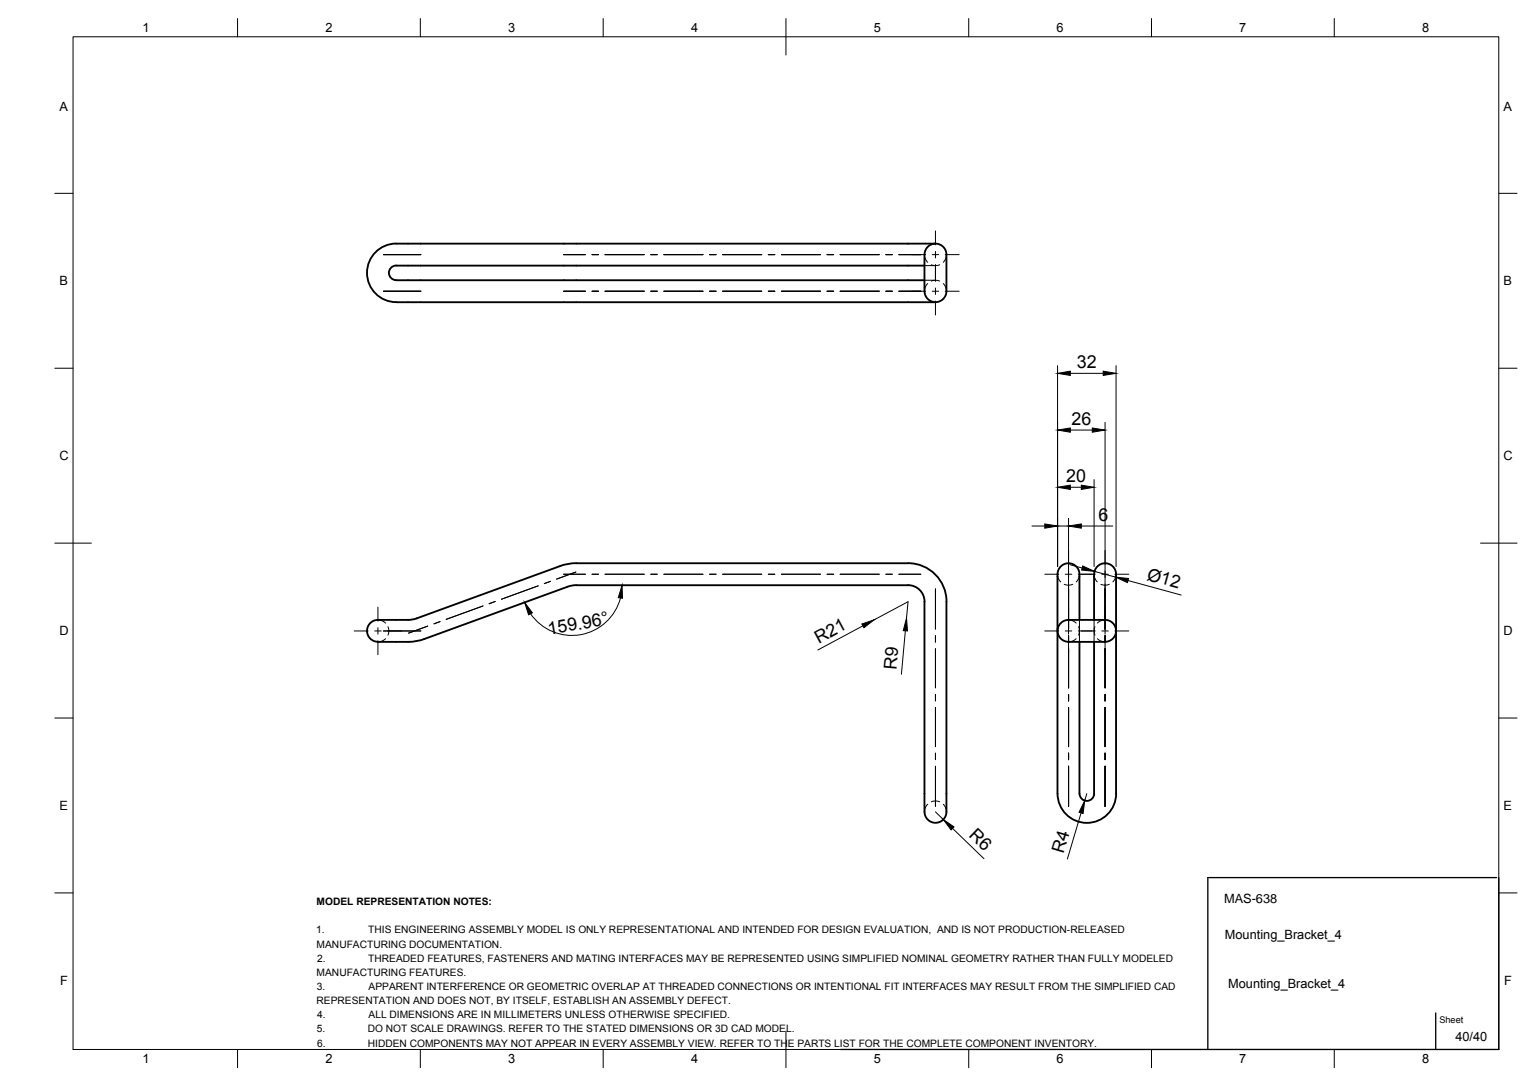
ISO-10303-21;
HEADER;
FILE_DESCRIPTION((''),'2;1');
FILE_NAME('Mounting_Bracket_4.step','2026-10-09T12:00:21-07:00',(''),(''),'','','');
FILE_SCHEMA (('AUTOMOTIVE_DESIGN { 1 0 10303 214 3 1 1 }'));
ENDSEC;
DATA;
#10=MECHANICAL_DESIGN_GEOMETRIC_PRESENTATION_REPRESENTATION('',(#435),#10334);
#184=CYLINDRICAL_SURFACE('',#4428,0.600000000000001) ;
#185=CYLINDRICAL_SURFACE('',#4429,0.600000000000001) ;
#186=CYLINDRICAL_SURFACE('',#4430,0.599999999999996) ;
#187=CYLINDRICAL_SURFACE('',#4431,0.600000000000001) ;
#188=CYLINDRICAL_SURFACE('',#4432,0.600000000000001) ;
#189=CYLINDRICAL_SURFACE('',#4433,0.600000000000001) ;
#190=CYLINDRICAL_SURFACE('',#4434,0.599999999999996) ;
#191=CYLINDRICAL_SURFACE('',#4435,0.600000000000001) ;
#363=SHAPE_REPRESENTATION_RELATIONSHIP('SRR','None',#10481,#395) ;
#395=ADVANCED_BREP_SHAPE_REPRESENTATION('',(#467),#10333) ;
#435=STYLED_ITEM('',(#10631),#467) ;
#467=MANIFOLD_SOLID_BREP('Body1',#3589) ;
#682=LINE('',#10238,#840) ;
#683=LINE('',#10240,#841) ;
#684=LINE('',#10242,#842) ;
#685=LINE('',#10244,#843) ;
#686=LINE('',#10246,#844) ;
#687=LINE('',#10248,#845) ;
#688=LINE('',#10250,#846) ;
#689=LINE('',#10252,#847) ;
#840=VECTOR('',#5566,0.600000000000001) ;
#841=VECTOR('',#5569,0.600000000000001) ;
#842=VECTOR('',#5572,0.599999999999996) ;
#843=VECTOR('',#5575,0.600000000000001) ;
#844=VECTOR('',#5578,0.600000000000001) ;
#845=VECTOR('',#5581,0.600000000000001) ;
#846=VECTOR('',#5584,0.599999999999996) ;
#847=VECTOR('',#5587,0.600000000000001) ;
#1034=FACE_OUTER_BOUND('',#1242,.T.) ;
#1035=FACE_OUTER_BOUND('',#1243,.T.) ;
#1036=FACE_OUTER_BOUND('',#1244,.T.) ;
#1037=FACE_OUTER_BOUND('',#1245,.T.) ;
#1038=FACE_OUTER_BOUND('',#1246,.T.) ;
#1039=FACE_OUTER_BOUND('',#1247,.T.) ;
#1040=FACE_OUTER_BOUND('',#1248,.T.) ;
#1041=FACE_OUTER_BOUND('',#1249,.T.) ;
#1042=FACE_OUTER_BOUND('',#1250,.T.) ;
#1043=FACE_OUTER_BOUND('',#1251,.T.) ;
#1044=FACE_OUTER_BOUND('',#1252,.T.) ;
#1045=FACE_OUTER_BOUND('',#1253,.T.) ;
#1046=FACE_OUTER_BOUND('',#1254,.T.) ;
#1047=FACE_OUTER_BOUND('',#1255,.T.) ;
#1048=FACE_OUTER_BOUND('',#1256,.T.) ;
#1049=FACE_OUTER_BOUND('',#1257,.T.) ;
#1242=EDGE_LOOP('',(#3217,#3218,#3219,#3220,#3221)) ;
#1243=EDGE_LOOP('',(#3222,#3223,#3224,#3225)) ;
#1244=EDGE_LOOP('',(#3226,#3227,#3228,#3229,#3230,#3231)) ;
#1245=EDGE_LOOP('',(#3232,#3233,#3234,#3235,#3236,#3237)) ;
#1246=EDGE_LOOP('',(#3238,#3239,#3240,#3241,#3242,#3243)) ;
#1247=EDGE_LOOP('',(#3244,#3245,#3246,#3247,#3248)) ;
#1248=EDGE_LOOP('',(#3249,#3250,#3251,#3252)) ;
#1249=EDGE_LOOP('',(#3253,#3254,#3255,#3256,#3257,#3258)) ;
#1250=EDGE_LOOP('',(#3259,#3260,#3261,#3262,#3263,#3264)) ;
#1251=EDGE_LOOP('',(#3265,#3266,#3267,#3268)) ;
#1252=EDGE_LOOP('',(#3269,#3270,#3271,#3272,#3273)) ;
#1253=EDGE_LOOP('',(#3274,#3275,#3276,#3277,#3278,#3279)) ;
#1254=EDGE_LOOP('',(#3280,#3281,#3282,#3283,#3284,#3285)) ;
#1255=EDGE_LOOP('',(#3286,#3287,#3288,#3289)) ;
#1256=EDGE_LOOP('',(#3290,#3291,#3292,#3293,#3294)) ;
#1257=EDGE_LOOP('',(#3295,#3296,#3297,#3298,#3299,#3300)) ;
#1465=CIRCLE('',#4387,0.600000000000001) ;
#1466=CIRCLE('',#4388,0.899999999999999) ;
#1467=CIRCLE('',#4389,0.600000000000001) ;
#1468=CIRCLE('',#4390,0.600000000000001) ;
#1469=CIRCLE('',#4392,0.600000000000001) ;
#1470=CIRCLE('',#4393,1.4) ;
#1471=CIRCLE('',#4394,0.600000000000001) ;
#1472=CIRCLE('',#4396,0.600000000000001) ;
#1473=CIRCLE('',#4397,0.600000000000001) ;
#1474=CIRCLE('',#4398,1.4) ;
#1475=CIRCLE('',#4399,0.600000000000001) ;
#1476=CIRCLE('',#4400,0.600000000000001) ;
#1477=CIRCLE('',#4402,0.600000000000001) ;
#1478=CIRCLE('',#4403,0.399999999999999) ;
#1479=CIRCLE('',#4404,0.600000000000001) ;
#1480=CIRCLE('',#4405,0.600000000000001) ;
#1481=CIRCLE('',#4406,0.600000000000001) ;
#1482=CIRCLE('',#4408,0.600000000000001) ;
#1483=CIRCLE('',#4409,0.600000000000001) ;
#1484=CIRCLE('',#4410,0.400000000000002) ;
#1485=CIRCLE('',#4411,0.600000000000001) ;
#1486=CIRCLE('',#4412,0.600000000000001) ;
#1487=CIRCLE('',#4414,0.600000000000001) ;
#1488=CIRCLE('',#4415,0.600000000000001) ;
#1489=CIRCLE('',#4416,0.899999999999999) ;
#1490=CIRCLE('',#4417,0.600000000000001) ;
#1491=CIRCLE('',#4419,0.600000000000001) ;
#1492=CIRCLE('',#4420,1.4) ;
#1493=CIRCLE('',#4421,0.600000000000001) ;
#1494=CIRCLE('',#4423,0.600000000000001) ;
#1495=CIRCLE('',#4424,0.600000000000001) ;
#1496=CIRCLE('',#4425,1.4) ;
#1497=CIRCLE('',#4426,0.600000000000001) ;
#1498=CIRCLE('',#4427,0.600000000000001) ;
#1784=VERTEX_POINT('',#10170) ;
#1785=VERTEX_POINT('',#10172) ;
#1786=VERTEX_POINT('',#10174) ;
#1787=VERTEX_POINT('',#10178) ;
#1788=VERTEX_POINT('',#10180) ;
#1789=VERTEX_POINT('',#10184) ;
#1790=VERTEX_POINT('',#10185) ;
#1791=VERTEX_POINT('',#10188) ;
#1792=VERTEX_POINT('',#10190) ;
#1793=VERTEX_POINT('',#10194) ;
#1794=VERTEX_POINT('',#10195) ;
#1795=VERTEX_POINT('',#10197) ;
#1796=VERTEX_POINT('',#10199) ;
#1797=VERTEX_POINT('',#10204) ;
#1798=VERTEX_POINT('',#10205) ;
#1799=VERTEX_POINT('',#10208) ;
#1800=VERTEX_POINT('',#10210) ;
#1801=VERTEX_POINT('',#10214) ;
#1802=VERTEX_POINT('',#10215) ;
#1803=VERTEX_POINT('',#10218) ;
#1804=VERTEX_POINT('',#10222) ;
#1805=VERTEX_POINT('',#10224) ;
#1806=VERTEX_POINT('',#10228) ;
#1807=VERTEX_POINT('',#10229) ;
#1808=VERTEX_POINT('',#10232) ;
#1809=VERTEX_POINT('',#10234) ;
#2265=EDGE_CURVE('',#1784,#1784,#1465,.T.) ;
#2266=EDGE_CURVE('',#1784,#1785,#1466,.T.) ;
#2267=EDGE_CURVE('',#1785,#1786,#1467,.T.) ;
#2268=EDGE_CURVE('',#1786,#1785,#1468,.T.) ;
#2269=EDGE_CURVE('',#1787,#1787,#1469,.T.) ;
#2270=EDGE_CURVE('',#1787,#1788,#1470,.T.) ;
#2271=EDGE_CURVE('',#1788,#1788,#1471,.T.) ;
#2272=EDGE_CURVE('',#1789,#1790,#1472,.T.) ;
#2273=EDGE_CURVE('',#1790,#1789,#1473,.T.) ;
#2274=EDGE_CURVE('',#1790,#1791,#1474,.T.) ;
#2275=EDGE_CURVE('',#1791,#1792,#1475,.T.) ;
#2276=EDGE_CURVE('',#1792,#1791,#1476,.T.) ;
#2277=EDGE_CURVE('',#1793,#1794,#1477,.T.) ;
#2278=EDGE_CURVE('',#1794,#1795,#1478,.T.) ;
#2279=EDGE_CURVE('',#1796,#1795,#1479,.T.) ;
#2280=EDGE_CURVE('',#1795,#1796,#1480,.T.) ;
#2281=EDGE_CURVE('',#1794,#1793,#1481,.T.) ;
#2282=EDGE_CURVE('',#1797,#1798,#1482,.T.) ;
#2283=EDGE_CURVE('',#1798,#1797,#1483,.T.) ;
#2284=EDGE_CURVE('',#1798,#1799,#1484,.T.) ;
#2285=EDGE_CURVE('',#1799,#1800,#1485,.T.) ;
#2286=EDGE_CURVE('',#1800,#1799,#1486,.T.) ;
#2287=EDGE_CURVE('',#1801,#1802,#1487,.T.) ;
#2288=EDGE_CURVE('',#1802,#1801,#1488,.T.) ;
#2289=EDGE_CURVE('',#1802,#1803,#1489,.T.) ;
#2290=EDGE_CURVE('',#1803,#1803,#1490,.T.) ;
#2291=EDGE_CURVE('',#1804,#1804,#1491,.T.) ;
#2292=EDGE_CURVE('',#1804,#1805,#1492,.T.) ;
#2293=EDGE_CURVE('',#1805,#1805,#1493,.T.) ;
#2294=EDGE_CURVE('',#1806,#1807,#1494,.T.) ;
#2295=EDGE_CURVE('',#1807,#1806,#1495,.T.) ;
#2296=EDGE_CURVE('',#1807,#1808,#1496,.T.) ;
#2297=EDGE_CURVE('',#1808,#1809,#1497,.T.) ;
#2298=EDGE_CURVE('',#1809,#1808,#1498,.T.) ;
#2299=EDGE_CURVE('',#1797,#1786,#682,.T.) ;
#2300=EDGE_CURVE('',#1784,#1788,#683,.T.) ;
#2301=EDGE_CURVE('',#1787,#1792,#684,.T.) ;
#2302=EDGE_CURVE('',#1789,#1793,#685,.T.) ;
#2303=EDGE_CURVE('',#1800,#1801,#686,.T.) ;
#2304=EDGE_CURVE('',#1803,#1804,#687,.T.) ;
#2305=EDGE_CURVE('',#1805,#1806,#688,.T.) ;
#2306=EDGE_CURVE('',#1809,#1796,#689,.T.) ;
#3217=ORIENTED_EDGE('',*,*,#2265,.F.) ;
#3218=ORIENTED_EDGE('',*,*,#2266,.T.) ;
#3219=ORIENTED_EDGE('',*,*,#2267,.T.) ;
#3220=ORIENTED_EDGE('',*,*,#2268,.T.) ;
#3221=ORIENTED_EDGE('',*,*,#2266,.F.) ;
#3222=ORIENTED_EDGE('',*,*,#2269,.F.) ;
#3223=ORIENTED_EDGE('',*,*,#2270,.T.) ;
#3224=ORIENTED_EDGE('',*,*,#2271,.T.) ;
#3225=ORIENTED_EDGE('',*,*,#2270,.F.) ;
#3226=ORIENTED_EDGE('',*,*,#2272,.F.) ;
#3227=ORIENTED_EDGE('',*,*,#2273,.F.) ;
#3228=ORIENTED_EDGE('',*,*,#2274,.T.) ;
#3229=ORIENTED_EDGE('',*,*,#2275,.T.) ;
#3230=ORIENTED_EDGE('',*,*,#2276,.T.) ;
#3231=ORIENTED_EDGE('',*,*,#2274,.F.) ;
#3232=ORIENTED_EDGE('',*,*,#2277,.T.) ;
#3233=ORIENTED_EDGE('',*,*,#2278,.T.) ;
#3234=ORIENTED_EDGE('',*,*,#2279,.F.) ;
#3235=ORIENTED_EDGE('',*,*,#2280,.F.) ;
#3236=ORIENTED_EDGE('',*,*,#2278,.F.) ;
#3237=ORIENTED_EDGE('',*,*,#2281,.T.) ;
#3238=ORIENTED_EDGE('',*,*,#2282,.F.) ;
#3239=ORIENTED_EDGE('',*,*,#2283,.F.) ;
#3240=ORIENTED_EDGE('',*,*,#2284,.T.) ;
#3241=ORIENTED_EDGE('',*,*,#2285,.T.) ;
#3242=ORIENTED_EDGE('',*,*,#2286,.T.) ;
#3243=ORIENTED_EDGE('',*,*,#2284,.F.) ;
#3244=ORIENTED_EDGE('',*,*,#2287,.F.) ;
#3245=ORIENTED_EDGE('',*,*,#2288,.F.) ;
#3246=ORIENTED_EDGE('',*,*,#2289,.T.) ;
#3247=ORIENTED_EDGE('',*,*,#2290,.T.) ;
#3248=ORIENTED_EDGE('',*,*,#2289,.F.) ;
#3249=ORIENTED_EDGE('',*,*,#2291,.F.) ;
#3250=ORIENTED_EDGE('',*,*,#2292,.T.) ;
#3251=ORIENTED_EDGE('',*,*,#2293,.T.) ;
#3252=ORIENTED_EDGE('',*,*,#2292,.F.) ;
#3253=ORIENTED_EDGE('',*,*,#2294,.F.) ;
#3254=ORIENTED_EDGE('',*,*,#2295,.F.) ;
#3255=ORIENTED_EDGE('',*,*,#2296,.T.) ;
#3256=ORIENTED_EDGE('',*,*,#2297,.T.) ;
#3257=ORIENTED_EDGE('',*,*,#2298,.T.) ;
#3258=ORIENTED_EDGE('',*,*,#2296,.F.) ;
#3259=ORIENTED_EDGE('',*,*,#2282,.T.) ;
#3260=ORIENTED_EDGE('',*,*,#2283,.T.) ;
#3261=ORIENTED_EDGE('',*,*,#2299,.T.) ;
#3262=ORIENTED_EDGE('',*,*,#2267,.F.) ;
#3263=ORIENTED_EDGE('',*,*,#2268,.F.) ;
#3264=ORIENTED_EDGE('',*,*,#2299,.F.) ;
#3265=ORIENTED_EDGE('',*,*,#2265,.T.) ;
#3266=ORIENTED_EDGE('',*,*,#2300,.T.) ;
#3267=ORIENTED_EDGE('',*,*,#2271,.F.) ;
#3268=ORIENTED_EDGE('',*,*,#2300,.F.) ;
#3269=ORIENTED_EDGE('',*,*,#2269,.T.) ;
#3270=ORIENTED_EDGE('',*,*,#2301,.T.) ;
#3271=ORIENTED_EDGE('',*,*,#2275,.F.) ;
#3272=ORIENTED_EDGE('',*,*,#2276,.F.) ;
#3273=ORIENTED_EDGE('',*,*,#2301,.F.) ;
#3274=ORIENTED_EDGE('',*,*,#2272,.T.) ;
#3275=ORIENTED_EDGE('',*,*,#2273,.T.) ;
#3276=ORIENTED_EDGE('',*,*,#2302,.T.) ;
#3277=ORIENTED_EDGE('',*,*,#2281,.F.) ;
#3278=ORIENTED_EDGE('',*,*,#2277,.F.) ;
#3279=ORIENTED_EDGE('',*,*,#2302,.F.) ;
#3280=ORIENTED_EDGE('',*,*,#2286,.F.) ;
#3281=ORIENTED_EDGE('',*,*,#2303,.T.) ;
#3282=ORIENTED_EDGE('',*,*,#2287,.T.) ;
#3283=ORIENTED_EDGE('',*,*,#2288,.T.) ;
#3284=ORIENTED_EDGE('',*,*,#2303,.F.) ;
#3285=ORIENTED_EDGE('',*,*,#2285,.F.) ;
#3286=ORIENTED_EDGE('',*,*,#2290,.F.) ;
#3287=ORIENTED_EDGE('',*,*,#2304,.T.) ;
#3288=ORIENTED_EDGE('',*,*,#2291,.T.) ;
#3289=ORIENTED_EDGE('',*,*,#2304,.F.) ;
#3290=ORIENTED_EDGE('',*,*,#2293,.F.) ;
#3291=ORIENTED_EDGE('',*,*,#2305,.T.) ;
#3292=ORIENTED_EDGE('',*,*,#2294,.T.) ;
#3293=ORIENTED_EDGE('',*,*,#2295,.T.) ;
#3294=ORIENTED_EDGE('',*,*,#2305,.F.) ;
#3295=ORIENTED_EDGE('',*,*,#2298,.F.) ;
#3296=ORIENTED_EDGE('',*,*,#2306,.T.) ;
#3297=ORIENTED_EDGE('',*,*,#2279,.T.) ;
#3298=ORIENTED_EDGE('',*,*,#2280,.T.) ;
#3299=ORIENTED_EDGE('',*,*,#2306,.F.) ;
#3300=ORIENTED_EDGE('',*,*,#2297,.F.) ;
#3351=TOROIDAL_SURFACE('',#4386,1.5,0.6) ;
#3352=TOROIDAL_SURFACE('',#4391,2.,0.6) ;
#3353=TOROIDAL_SURFACE('',#4395,2.,0.6) ;
#3354=TOROIDAL_SURFACE('',#4401,1.,0.6) ;
#3355=TOROIDAL_SURFACE('',#4407,1.,0.599999999999999) ;
#3356=TOROIDAL_SURFACE('',#4413,1.5,0.6) ;
#3357=TOROIDAL_SURFACE('',#4418,2.,0.6) ;
#3358=TOROIDAL_SURFACE('',#4422,2.,0.6) ;
#3542=ADVANCED_FACE('',(#1034),#3351,.T.) ;
#3543=ADVANCED_FACE('',(#1035),#3352,.T.) ;
#3544=ADVANCED_FACE('',(#1036),#3353,.T.) ;
#3545=ADVANCED_FACE('',(#1037),#3354,.T.) ;
#3546=ADVANCED_FACE('',(#1038),#3355,.T.) ;
#3547=ADVANCED_FACE('',(#1039),#3356,.T.) ;
#3548=ADVANCED_FACE('',(#1040),#3357,.T.) ;
#3549=ADVANCED_FACE('',(#1041),#3358,.T.) ;
#3550=ADVANCED_FACE('',(#1042),#184,.T.) ;
#3551=ADVANCED_FACE('',(#1043),#185,.T.) ;
#3552=ADVANCED_FACE('',(#1044),#186,.T.) ;
#3553=ADVANCED_FACE('',(#1045),#187,.T.) ;
#3554=ADVANCED_FACE('',(#1046),#188,.T.) ;
#3555=ADVANCED_FACE('',(#1047),#189,.T.) ;
#3556=ADVANCED_FACE('',(#1048),#190,.T.) ;
#3557=ADVANCED_FACE('',(#1049),#191,.T.) ;
#3589=CLOSED_SHELL('',(#3542,#3543,#3544,#3545,#3546,#3547,#3548,#3549,
#3550,#3551,#3552,#3553,#3554,#3555,#3556,#3557)) ;
#4385=AXIS2_PLACEMENT_3D('',#10168,#5478,#5479) ;
#4386=AXIS2_PLACEMENT_3D('',#10169,#5480,#5481) ;
#4387=AXIS2_PLACEMENT_3D('',#10171,#5482,#5483) ;
#4388=AXIS2_PLACEMENT_3D('',#10173,#5484,#5485) ;
#4389=AXIS2_PLACEMENT_3D('',#10175,#5486,#5487) ;
#4390=AXIS2_PLACEMENT_3D('',#10176,#5488,#5489) ;
#4391=AXIS2_PLACEMENT_3D('',#10177,#5490,#5491) ;
#4392=AXIS2_PLACEMENT_3D('',#10179,#5492,#5493) ;
#4393=AXIS2_PLACEMENT_3D('',#10181,#5494,#5495) ;
#4394=AXIS2_PLACEMENT_3D('',#10182,#5496,#5497) ;
#4395=AXIS2_PLACEMENT_3D('',#10183,#5498,#5499) ;
#4396=AXIS2_PLACEMENT_3D('',#10186,#5500,#5501) ;
#4397=AXIS2_PLACEMENT_3D('',#10187,#5502,#5503) ;
#4398=AXIS2_PLACEMENT_3D('',#10189,#5504,#5505) ;
#4399=AXIS2_PLACEMENT_3D('',#10191,#5506,#5507) ;
#4400=AXIS2_PLACEMENT_3D('',#10192,#5508,#5509) ;
#4401=AXIS2_PLACEMENT_3D('',#10193,#5510,#5511) ;
#4402=AXIS2_PLACEMENT_3D('',#10196,#5512,#5513) ;
#4403=AXIS2_PLACEMENT_3D('',#10198,#5514,#5515) ;
#4404=AXIS2_PLACEMENT_3D('',#10200,#5516,#5517) ;
#4405=AXIS2_PLACEMENT_3D('',#10201,#5518,#5519) ;
#4406=AXIS2_PLACEMENT_3D('',#10202,#5520,#5521) ;
#4407=AXIS2_PLACEMENT_3D('',#10203,#5522,#5523) ;
#4408=AXIS2_PLACEMENT_3D('',#10206,#5524,#5525) ;
#4409=AXIS2_PLACEMENT_3D('',#10207,#5526,#5527) ;
#4410=AXIS2_PLACEMENT_3D('',#10209,#5528,#5529) ;
#4411=AXIS2_PLACEMENT_3D('',#10211,#5530,#5531) ;
#4412=AXIS2_PLACEMENT_3D('',#10212,#5532,#5533) ;
#4413=AXIS2_PLACEMENT_3D('',#10213,#5534,#5535) ;
#4414=AXIS2_PLACEMENT_3D('',#10216,#5536,#5537) ;
#4415=AXIS2_PLACEMENT_3D('',#10217,#5538,#5539) ;
#4416=AXIS2_PLACEMENT_3D('',#10219,#5540,#5541) ;
#4417=AXIS2_PLACEMENT_3D('',#10220,#5542,#5543) ;
#4418=AXIS2_PLACEMENT_3D('',#10221,#5544,#5545) ;
#4419=AXIS2_PLACEMENT_3D('',#10223,#5546,#5547) ;
#4420=AXIS2_PLACEMENT_3D('',#10225,#5548,#5549) ;
#4421=AXIS2_PLACEMENT_3D('',#10226,#5550,#5551) ;
#4422=AXIS2_PLACEMENT_3D('',#10227,#5552,#5553) ;
#4423=AXIS2_PLACEMENT_3D('',#10230,#5554,#5555) ;
#4424=AXIS2_PLACEMENT_3D('',#10231,#5556,#5557) ;
#4425=AXIS2_PLACEMENT_3D('',#10233,#5558,#5559) ;
#4426=AXIS2_PLACEMENT_3D('',#10235,#5560,#5561) ;
#4427=AXIS2_PLACEMENT_3D('',#10236,#5562,#5563) ;
#4428=AXIS2_PLACEMENT_3D('',#10237,#5564,#5565) ;
#4429=AXIS2_PLACEMENT_3D('',#10239,#5567,#5568) ;
#4430=AXIS2_PLACEMENT_3D('',#10241,#5570,#5571) ;
#4431=AXIS2_PLACEMENT_3D('',#10243,#5573,#5574) ;
#4432=AXIS2_PLACEMENT_3D('',#10245,#5576,#5577) ;
#4433=AXIS2_PLACEMENT_3D('',#10247,#5579,#5580) ;
#4434=AXIS2_PLACEMENT_3D('',#10249,#5582,#5583) ;
#4435=AXIS2_PLACEMENT_3D('',#10251,#5585,#5586) ;
#5478=DIRECTION('axis',(0.,0.,1.)) ;
#5479=DIRECTION('refdir',(1.,0.,0.)) ;
#5480=DIRECTION('center_axis',(1.,0.,1.03724286811635E-14)) ;
#5481=DIRECTION('ref_axis',(-1.01506105108586E-14,0.,1.)) ;
#5482=DIRECTION('center_axis',(-1.03724286811635E-14,0.,1.)) ;
#5483=DIRECTION('ref_axis',(1.,0.,1.03724286811635E-14)) ;
#5484=DIRECTION('center_axis',(-1.,0.,-1.03724286811635E-14)) ;
#5485=DIRECTION('ref_axis',(-1.03724286811635E-14,0.,1.)) ;
#5486=DIRECTION('center_axis',(0.,1.,0.)) ;
#5487=DIRECTION('ref_axis',(1.,0.,9.25185853854296E-15)) ;
#5488=DIRECTION('center_axis',(0.,1.,0.)) ;
#5489=DIRECTION('ref_axis',(1.,0.,9.25185853854296E-15)) ;
#5490=DIRECTION('center_axis',(1.,0.,1.03724286811635E-14)) ;
#5491=DIRECTION('ref_axis',(-1.09314267040015E-14,0.,1.)) ;
#5492=DIRECTION('center_axis',(-9.74458869605016E-15,-0.342630345100702,
0.93947030108257)) ;
#5493=DIRECTION('ref_axis',(1.,2.61738882522057E-15,1.13270057821263E-14)) ;
#5494=DIRECTION('center_axis',(-1.,0.,-1.03724286811635E-14)) ;
#5495=DIRECTION('ref_axis',(-1.03724286811635E-14,0.,1.)) ;
#5496=DIRECTION('center_axis',(-1.03724286811635E-14,0.,1.)) ;
#5497=DIRECTION('ref_axis',(1.,0.,1.03724286811635E-14)) ;
#5498=DIRECTION('center_axis',(-1.,0.,-1.03724286811635E-14)) ;
#5499=DIRECTION('ref_axis',(1.09314267040015E-14,0.,-1.)) ;
#5500=DIRECTION('center_axis',(-1.03724286811635E-14,0.,1.)) ;
#5501=DIRECTION('ref_axis',(1.,0.,1.03724286811635E-14)) ;
#5502=DIRECTION('center_axis',(-1.03724286811635E-14,0.,1.)) ;
#5503=DIRECTION('ref_axis',(1.,0.,1.03724286811635E-14)) ;
#5504=DIRECTION('center_axis',(1.,0.,1.03724286811635E-14)) ;
#5505=DIRECTION('ref_axis',(1.03724286811635E-14,0.,-1.)) ;
#5506=DIRECTION('center_axis',(-9.74458869605016E-15,-0.342630345100702,
0.93947030108257)) ;
#5507=DIRECTION('ref_axis',(1.,2.61738882522057E-15,1.13270057821263E-14)) ;
#5508=DIRECTION('center_axis',(-9.74458869605016E-15,-0.342630345100702,
0.93947030108257)) ;
#5509=DIRECTION('ref_axis',(1.,2.61738882522057E-15,1.13270057821263E-14)) ;
#5510=DIRECTION('center_axis',(0.,-1.,0.)) ;
#5511=DIRECTION('ref_axis',(-1.,0.,-1.33226762955019E-14)) ;
#5512=DIRECTION('center_axis',(-1.03724286811635E-14,0.,1.)) ;
#5513=DIRECTION('ref_axis',(1.,0.,1.03724286811635E-14)) ;
#5514=DIRECTION('center_axis',(0.,1.,0.)) ;
#5515=DIRECTION('ref_axis',(-1.,0.,-1.77635683940026E-14)) ;
#5516=DIRECTION('center_axis',(1.04744440165294E-14,0.,-1.)) ;
#5517=DIRECTION('ref_axis',(-1.,0.,-1.04744440165294E-14)) ;
#5518=DIRECTION('center_axis',(1.04744440165294E-14,0.,-1.)) ;
#5519=DIRECTION('ref_axis',(-1.,0.,-1.04744440165294E-14)) ;
#5520=DIRECTION('center_axis',(-1.03724286811635E-14,0.,1.)) ;
#5521=DIRECTION('ref_axis',(1.,0.,1.03724286811635E-14)) ;
#5522=DIRECTION('center_axis',(1.04744440165294E-14,0.,-1.)) ;
#5523=DIRECTION('ref_axis',(-1.,0.,-1.11022302462516E-14)) ;
#5524=DIRECTION('center_axis',(0.,1.,0.)) ;
#5525=DIRECTION('ref_axis',(1.,0.,9.25185853854296E-15)) ;
#5526=DIRECTION('center_axis',(0.,1.,0.)) ;
#5527=DIRECTION('ref_axis',(1.,0.,9.25185853854296E-15)) ;
#5528=DIRECTION('center_axis',(-1.04744440165294E-14,0.,1.)) ;
#5529=DIRECTION('ref_axis',(-1.,0.,-1.04744440165294E-14)) ;
#5530=DIRECTION('center_axis',(0.,-1.,0.)) ;
#5531=DIRECTION('ref_axis',(-1.,0.,-9.25185853854296E-15)) ;
#5532=DIRECTION('center_axis',(0.,-1.,0.)) ;
#5533=DIRECTION('ref_axis',(-1.,0.,-9.25185853854296E-15)) ;
#5534=DIRECTION('center_axis',(-1.,0.,-1.04744440165294E-14)) ;
#5535=DIRECTION('ref_axis',(-1.01506105108586E-14,0.,1.)) ;
#5536=DIRECTION('center_axis',(0.,-1.,0.)) ;
#5537=DIRECTION('ref_axis',(-1.,0.,-9.25185853854296E-15)) ;
#5538=DIRECTION('center_axis',(0.,-1.,0.)) ;
#5539=DIRECTION('ref_axis',(-1.,0.,-9.25185853854296E-15)) ;
#5540=DIRECTION('center_axis',(1.,0.,1.04744440165294E-14)) ;
#5541=DIRECTION('ref_axis',(-1.04744440165294E-14,0.,1.)) ;
#5542=DIRECTION('center_axis',(1.04744440165294E-14,0.,-1.)) ;
#5543=DIRECTION('ref_axis',(-1.,0.,-1.04744440165294E-14)) ;
#5544=DIRECTION('center_axis',(-1.,0.,-1.04744440165294E-14)) ;
#5545=DIRECTION('ref_axis',(-1.09314267040015E-14,0.,1.)) ;
#5546=DIRECTION('center_axis',(1.04744440165294E-14,0.,-1.)) ;
#5547=DIRECTION('ref_axis',(-1.,0.,-1.04744440165294E-14)) ;
#5548=DIRECTION('center_axis',(1.,0.,1.04744440165294E-14)) ;
#5549=DIRECTION('ref_axis',(-1.04744440165294E-14,0.,1.)) ;
#5550=DIRECTION('center_axis',(9.8404290738814E-15,0.342630345100702,-0.93947030108257)) ;
#5551=DIRECTION('ref_axis',(-1.,-2.58455100348968E-15,-1.14170449707433E-14)) ;
#5552=DIRECTION('center_axis',(1.,0.,1.04744440165294E-14)) ;
#5553=DIRECTION('ref_axis',(1.09314267040015E-14,0.,-1.)) ;
#5554=DIRECTION('center_axis',(9.8404290738814E-15,0.342630345100702,-0.93947030108257)) ;
#5555=DIRECTION('ref_axis',(-1.,-2.58455100348968E-15,-1.14170449707433E-14)) ;
#5556=DIRECTION('center_axis',(9.8404290738814E-15,0.342630345100702,-0.93947030108257)) ;
#5557=DIRECTION('ref_axis',(-1.,-2.58455100348968E-15,-1.14170449707433E-14)) ;
#5558=DIRECTION('center_axis',(-1.,0.,-1.04744440165294E-14)) ;
#5559=DIRECTION('ref_axis',(1.04744440165294E-14,0.,-1.)) ;
#5560=DIRECTION('center_axis',(1.04744440165294E-14,0.,-1.)) ;
#5561=DIRECTION('ref_axis',(-1.,0.,-1.04744440165294E-14)) ;
#5562=DIRECTION('center_axis',(1.04744440165294E-14,0.,-1.)) ;
#5563=DIRECTION('ref_axis',(-1.,0.,-1.04744440165294E-14)) ;
#5564=DIRECTION('center_axis',(0.,-1.,0.)) ;
#5565=DIRECTION('ref_axis',(1.,0.,9.25185853854296E-15)) ;
#5566=DIRECTION('',(0.,1.,0.)) ;
#5567=DIRECTION('center_axis',(1.03724286811635E-14,1.91189112624469E-17,
-1.)) ;
#5568=DIRECTION('ref_axis',(-1.98309543531224E-31,1.,1.91189112624469E-17)) ;
#5569=DIRECTION('',(-1.03724286811635E-14,-1.91189112624469E-17,1.)) ;
#5570=DIRECTION('center_axis',(9.74458869605016E-15,0.342630345100702,-0.93947030108257)) ;
#5571=DIRECTION('ref_axis',(-4.62592926927152E-15,0.93947030108257,0.342630345100702)) ;
#5572=DIRECTION('',(-9.74458869605016E-15,-0.342630345100702,0.93947030108257)) ;
#5573=DIRECTION('center_axis',(1.03724286811635E-14,0.,-1.)) ;
#5574=DIRECTION('ref_axis',(1.,0.,1.03724286811635E-14)) ;
#5575=DIRECTION('',(-1.03724286811635E-14,0.,1.)) ;
#5576=DIRECTION('center_axis',(0.,-1.,0.)) ;
#5577=DIRECTION('ref_axis',(-1.,0.,-9.25185853854296E-15)) ;
#5578=DIRECTION('',(0.,1.,0.)) ;
#5579=DIRECTION('center_axis',(1.04744440165294E-14,1.91189112624469E-17,
-1.)) ;
#5580=DIRECTION('ref_axis',(-2.00259965675493E-31,1.,1.91189112624469E-17)) ;
#5581=DIRECTION('',(-1.04744440165294E-14,-1.91189112624469E-17,1.)) ;
#5582=DIRECTION('center_axis',(9.8404290738814E-15,0.342630345100702,-0.93947030108257)) ;
#5583=DIRECTION('ref_axis',(-4.62592926927152E-15,0.93947030108257,0.342630345100702)) ;
#5584=DIRECTION('',(-9.8404290738814E-15,-0.342630345100702,0.93947030108257)) ;
#5585=DIRECTION('center_axis',(1.04744440165294E-14,0.,-1.)) ;
#5586=DIRECTION('ref_axis',(-1.,0.,-1.04744440165294E-14)) ;
#5587=DIRECTION('',(-1.04744440165294E-14,0.,1.)) ;
#10168=CARTESIAN_POINT('',(0.,0.,0.)) ;
#10169=CARTESIAN_POINT('Origin',(22.4776880157603,67.0830586252741,32.9724337400001)) ;
#10170=CARTESIAN_POINT('',(22.4776880157602,67.9830586252741,32.9724337400001)) ;
#10171=CARTESIAN_POINT('Origin',(22.4776880157603,68.5830586252741,32.9724337400001)) ;
#10172=CARTESIAN_POINT('',(22.4776880157603,67.0830586252741,32.0724337400002)) ;
#10173=CARTESIAN_POINT('Origin',(22.4776880157603,67.0830586252741,32.9724337400001)) ;
#10174=CARTESIAN_POINT('',(21.8776880157603,67.0830586252741,31.4724337400001)) ;
#10175=CARTESIAN_POINT('Origin',(22.4776880157603,67.0830586252741,31.4724337400002)) ;
#10176=CARTESIAN_POINT('Origin',(22.4776880157603,67.0830586252741,31.4724337400002)) ;
#10177=CARTESIAN_POINT('Origin',(22.4776880157601,66.5830586252741,51.1191101083782)) ;
#10178=CARTESIAN_POINT('',(22.4776880157601,67.8983170467897,51.5987925915192)) ;
#10179=CARTESIAN_POINT('Origin',(22.4776880157601,68.4619992274392,51.8043707985796)) ;
#10180=CARTESIAN_POINT('',(22.4776880157602,67.9830586252741,51.1191101083782)) ;
#10181=CARTESIAN_POINT('Origin',(22.4776880157601,66.5830586252741,51.1191101083782)) ;
#10182=CARTESIAN_POINT('Origin',(22.4776880157601,68.5830586252741,51.1191101083782)) ;
#10183=CARTESIAN_POINT('Origin',(22.47768801576,67.4830586252741,60.3257573716221)) ;
#10184=CARTESIAN_POINT('',(21.87768801576,65.4830586252741,60.3257573716221)) ;
#10185=CARTESIAN_POINT('',(22.47768801576,66.0830586252741,60.3257573716221)) ;
#10186=CARTESIAN_POINT('Origin',(22.47768801576,65.4830586252741,60.3257573716221)) ;
#10187=CARTESIAN_POINT('Origin',(22.47768801576,65.4830586252741,60.3257573716221)) ;
#10188=CARTESIAN_POINT('',(22.47768801576,66.1678002037585,59.8460748884811)) ;
#10189=CARTESIAN_POINT('Origin',(22.47768801576,67.4830586252741,60.3257573716221)) ;
#10190=CARTESIAN_POINT('',(22.47768801576,65.0404358424594,59.4349184743603)) ;
#10191=CARTESIAN_POINT('Origin',(22.47768801576,65.604118023109,59.6404966814207)) ;
#10192=CARTESIAN_POINT('Origin',(22.47768801576,65.604118023109,59.6404966814207)) ;
#10193=CARTESIAN_POINT('Origin',(23.47768801576,65.4830586252741,60.9724337400002)) ;
#10194=CARTESIAN_POINT('',(21.87768801576,65.4830586252741,60.9724337400001)) ;
#10195=CARTESIAN_POINT('',(23.07768801576,65.4830586252741,60.9724337400002)) ;
#10196=CARTESIAN_POINT('Origin',(22.47768801576,65.4830586252741,60.9724337400002)) ;
#10197=CARTESIAN_POINT('',(23.87768801576,65.4830586252741,60.9724337400002)) ;
#10198=CARTESIAN_POINT('Origin',(23.47768801576,65.4830586252741,60.9724337400002)) ;
#10199=CARTESIAN_POINT('',(25.07768801576,65.4830586252741,60.9724337400002)) ;
#10200=CARTESIAN_POINT('Origin',(24.47768801576,65.4830586252741,60.9724337400002)) ;
#10201=CARTESIAN_POINT('Origin',(24.47768801576,65.4830586252741,60.9724337400002)) ;
#10202=CARTESIAN_POINT('Origin',(22.47768801576,65.4830586252741,60.9724337400002)) ;
#10203=CARTESIAN_POINT('Origin',(23.4776880157603,56.5830586252741,31.4724337400002)) ;
#10204=CARTESIAN_POINT('',(21.8776880157603,56.5830586252741,31.4724337400001)) ;
#10205=CARTESIAN_POINT('',(23.0776880157603,56.5830586252741,31.4724337400002)) ;
#10206=CARTESIAN_POINT('Origin',(22.4776880157603,56.5830586252741,31.4724337400002)) ;
#10207=CARTESIAN_POINT('Origin',(22.4776880157603,56.5830586252741,31.4724337400002)) ;
#10208=CARTESIAN_POINT('',(23.8776880157603,56.5830586252741,31.4724337400002)) ;
#10209=CARTESIAN_POINT('Origin',(23.4776880157603,56.5830586252741,31.4724337400002)) ;
#10210=CARTESIAN_POINT('',(25.0776880157603,56.5830586252741,31.4724337400002)) ;
#10211=CARTESIAN_POINT('Origin',(24.4776880157603,56.5830586252741,31.4724337400002)) ;
#10212=CARTESIAN_POINT('Origin',(24.4776880157603,56.5830586252741,31.4724337400002)) ;
#10213=CARTESIAN_POINT('Origin',(24.4776880157603,67.0830586252741,32.9724337400002)) ;
#10214=CARTESIAN_POINT('',(25.0776880157603,67.0830586252741,31.4724337400002)) ;
#10215=CARTESIAN_POINT('',(24.4776880157603,67.0830586252741,32.0724337400002)) ;
#10216=CARTESIAN_POINT('Origin',(24.4776880157603,67.0830586252741,31.4724337400002)) ;
#10217=CARTESIAN_POINT('Origin',(24.4776880157603,67.0830586252741,31.4724337400002)) ;
#10218=CARTESIAN_POINT('',(24.4776880157602,67.9830586252741,32.9724337400002)) ;
#10219=CARTESIAN_POINT('Origin',(24.4776880157603,67.0830586252741,32.9724337400002)) ;
#10220=CARTESIAN_POINT('Origin',(24.4776880157603,68.5830586252741,32.9724337400002)) ;
#10221=CARTESIAN_POINT('Origin',(24.4776880157601,66.5830586252741,51.1191101083782)) ;
#10222=CARTESIAN_POINT('',(24.4776880157602,67.9830586252741,51.1191101083782)) ;
#10223=CARTESIAN_POINT('Origin',(24.4776880157601,68.5830586252741,51.1191101083782)) ;
#10224=CARTESIAN_POINT('',(24.4776880157601,67.8983170467897,51.5987925915192)) ;
#10225=CARTESIAN_POINT('Origin',(24.4776880157601,66.5830586252741,51.1191101083782)) ;
#10226=CARTESIAN_POINT('Origin',(24.4776880157601,68.4619992274392,51.8043707985796)) ;
#10227=CARTESIAN_POINT('Origin',(24.47768801576,67.4830586252741,60.3257573716221)) ;
#10228=CARTESIAN_POINT('',(24.47768801576,65.0404358424594,59.4349184743603)) ;
#10229=CARTESIAN_POINT('',(24.47768801576,66.1678002037585,59.8460748884811)) ;
#10230=CARTESIAN_POINT('Origin',(24.47768801576,65.604118023109,59.6404966814207)) ;
#10231=CARTESIAN_POINT('Origin',(24.47768801576,65.604118023109,59.6404966814207)) ;
#10232=CARTESIAN_POINT('',(24.47768801576,66.0830586252741,60.3257573716221)) ;
#10233=CARTESIAN_POINT('Origin',(24.47768801576,67.4830586252741,60.3257573716221)) ;
#10234=CARTESIAN_POINT('',(25.07768801576,65.4830586252741,60.3257573716221)) ;
#10235=CARTESIAN_POINT('Origin',(24.47768801576,65.4830586252741,60.3257573716221)) ;
#10236=CARTESIAN_POINT('Origin',(24.47768801576,65.4830586252741,60.3257573716221)) ;
#10237=CARTESIAN_POINT('Origin',(22.4776880157603,67.0830586252741,31.4724337400002)) ;
#10238=CARTESIAN_POINT('',(21.8776880157603,67.0830586252741,31.4724337400002)) ;
#10239=CARTESIAN_POINT('Origin',(22.4776880157601,68.5830586252741,51.1191101083782)) ;
#10240=CARTESIAN_POINT('',(22.4776880157601,67.9830586252741,51.1191101083782)) ;
#10241=CARTESIAN_POINT('Origin',(22.47768801576,65.6041180231089,59.6404966814207)) ;
#10242=CARTESIAN_POINT('',(22.47768801576,65.0404358424594,59.4349184743603)) ;
#10243=CARTESIAN_POINT('Origin',(22.47768801576,65.4830586252741,60.9724337400002)) ;
#10244=CARTESIAN_POINT('',(21.87768801576,65.4830586252741,60.9724337400002)) ;
#10245=CARTESIAN_POINT('Origin',(24.4776880157603,67.0830586252741,31.4724337400002)) ;
#10246=CARTESIAN_POINT('',(25.0776880157603,67.0830586252741,31.4724337400002)) ;
#10247=CARTESIAN_POINT('Origin',(24.4776880157601,68.5830586252741,51.1191101083782)) ;
#10248=CARTESIAN_POINT('',(24.4776880157601,67.9830586252741,51.1191101083782)) ;
#10249=CARTESIAN_POINT('Origin',(24.47768801576,65.6041180231089,59.6404966814207)) ;
#10250=CARTESIAN_POINT('',(24.47768801576,65.0404358424594,59.4349184743603)) ;
#10251=CARTESIAN_POINT('Origin',(24.47768801576,65.4830586252741,60.9724337400002)) ;
#10252=CARTESIAN_POINT('',(25.07768801576,65.4830586252741,60.9724337400002)) ;
#10296=UNCERTAINTY_MEASURE_WITH_UNIT(LENGTH_MEASURE(0.001),#10335,
'DISTANCE_ACCURACY_VALUE',
'Maximum model space distance between geometric entities at asserted c
onnectivities') ;
#10297=UNCERTAINTY_MEASURE_WITH_UNIT(LENGTH_MEASURE(0.001),#10335,
'DISTANCE_ACCURACY_VALUE',
'Maximum model space distance between geometric entities at asserted c
onnectivities') ;
#10333=(
GEOMETRIC_REPRESENTATION_CONTEXT(3)
GLOBAL_UNCERTAINTY_ASSIGNED_CONTEXT((#10296))
GLOBAL_UNIT_ASSIGNED_CONTEXT((#10335,#10337,#10338))
REPRESENTATION_CONTEXT('','3D')
) ;
#10334=(
GEOMETRIC_REPRESENTATION_CONTEXT(3)
GLOBAL_UNCERTAINTY_ASSIGNED_CONTEXT((#10297))
GLOBAL_UNIT_ASSIGNED_CONTEXT((#10335,#10337,#10338))
REPRESENTATION_CONTEXT('','3D')
) ;
#10335=(
LENGTH_UNIT()
NAMED_UNIT(*)
SI_UNIT(.CENTI.,.METRE.)
) ;
#10337=(
NAMED_UNIT(*)
PLANE_ANGLE_UNIT()
SI_UNIT($,.RADIAN.)
) ;
#10338=(
NAMED_UNIT(*)
SI_UNIT($,.STERADIAN.)
SOLID_ANGLE_UNIT()
) ;
#10374=SHAPE_DEFINITION_REPRESENTATION(#10437,#10481) ;
#10437=PRODUCT_DEFINITION_SHAPE('',$,#10518) ;
#10481=SHAPE_REPRESENTATION('',(#4385),#10333) ;
#10482=PRODUCT_DEFINITION_CONTEXT('part definition',#10592,'design') ;
#10518=PRODUCT_DEFINITION('Mounting_Bracket_4','Mounting_Bracket_4',#10554,
#10482) ;
#10554=PRODUCT_DEFINITION_FORMATION('',$,#10629) ;
#10592=APPLICATION_CONTEXT(
'Core Data for Automotive Mechanical Design Process') ;
#10593=PRODUCT_CONTEXT('part definition',#10592,'mechanical') ;
#10629=PRODUCT('Mounting_Bracket_4','Mounting_Bracket_4',$,(#10593)) ;
#10631=PRESENTATION_STYLE_ASSIGNMENT((#10635)) ;
#10635=SURFACE_STYLE_USAGE(.BOTH.,#10639) ;
#10639=SURFACE_SIDE_STYLE('',(#10643)) ;
#10643=SURFACE_STYLE_FILL_AREA(#10647) ;
#10647=FILL_AREA_STYLE('Opaque(25,25,25)',(#10651)) ;
#10651=FILL_AREA_STYLE_COLOUR('Opaque(25,25,25)',#10655) ;
#10655=COLOUR_RGB('Opaque(25,25,25)', 0.09019608, 0.27058824, 0.51372549) ;
ENDSEC;
END-ISO-10303-21;
